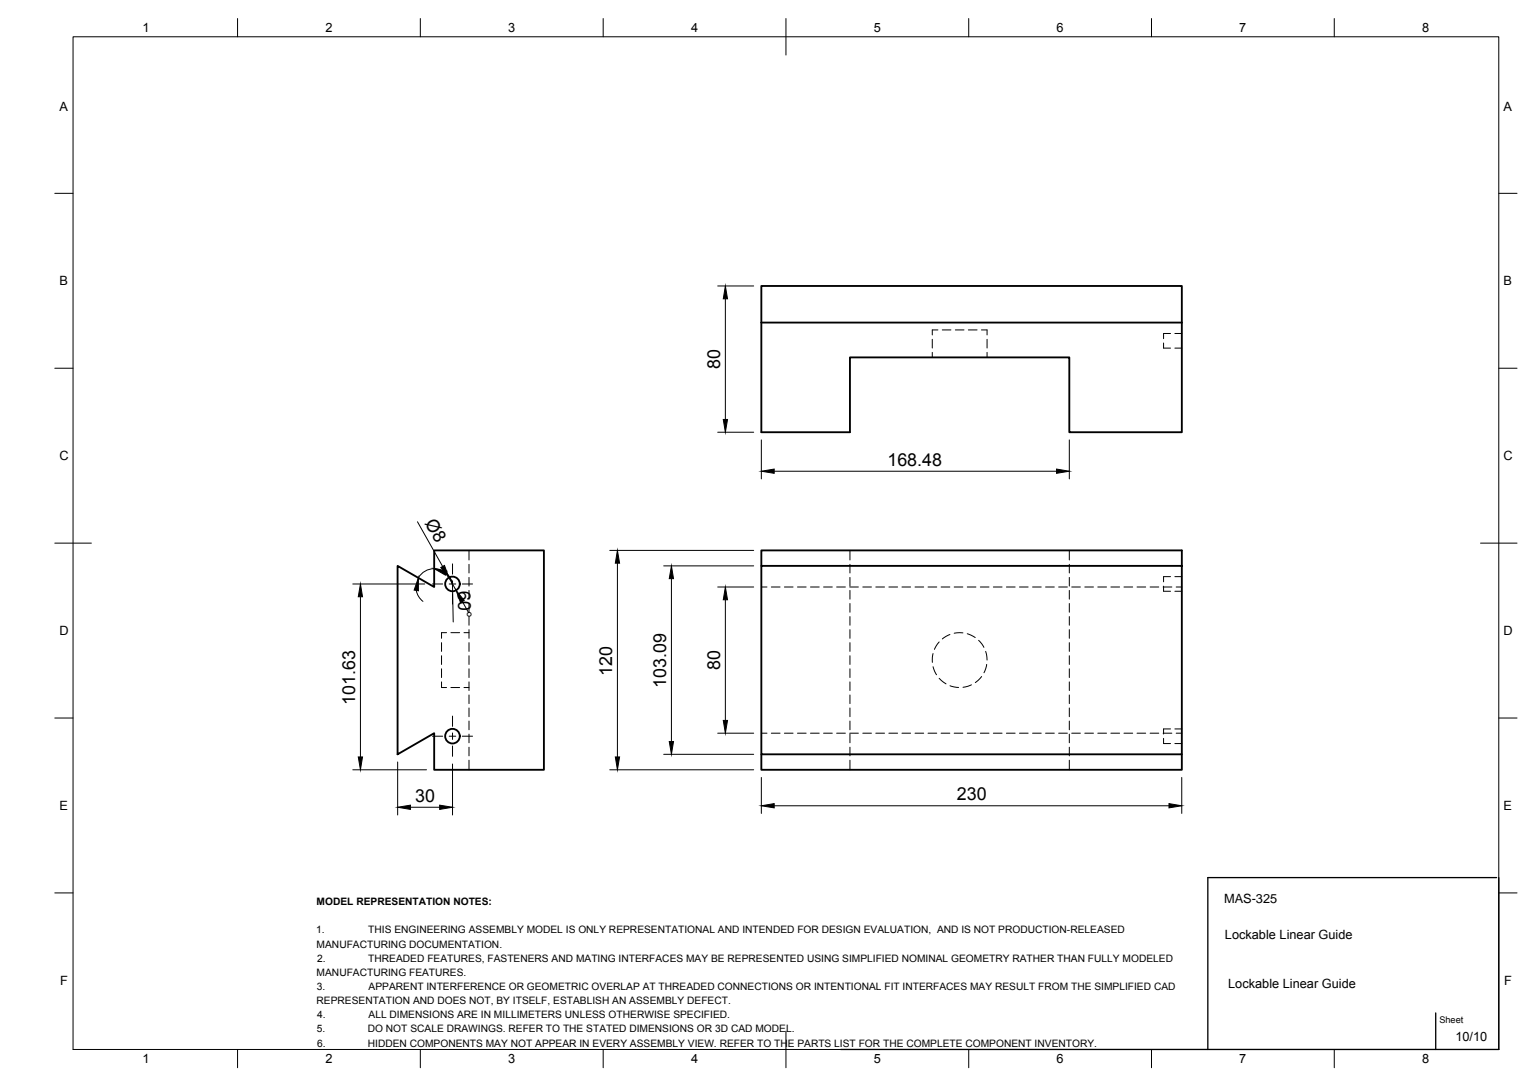
ISO-10303-21;
HEADER;
FILE_DESCRIPTION (('STEP AP214'),
    '1' );
FILE_NAME ('Lockable Linear Guide.step',
    '2026-10-08T01:23:29',
    ( '' ),
    ( '' ),
    'SwSTEP 2.0',
    'SolidWorks 2025',
    '' );
FILE_SCHEMA (( 'AUTOMOTIVE_DESIGN' ));
ENDSEC;

DATA;
#90=ORIENTED_EDGE ( 'NONE', *, *, #2858, .T. ) ;
#132=EDGE_LOOP ( 'NONE', ( #26426, #7526, #45933, #33902, #50296, #18073, #41197, #48921 ) ) ;
#156=DIRECTION ( 'NONE',  ( -1.000000000000000000, 0.000000000000000000, 0.000000000000000000 ) ) ;
#179=CIRCLE ( 'NONE', #49719, 4.000000000000003553 ) ;
#250=EDGE_CURVE ( 'NONE', #5889, #26611, #27078, .T. ) ;
#277=CARTESIAN_POINT ( 'NONE',  ( -108.4791267515088435, -173.5000000000000284, 60.00000000000002132 ) ) ;
#336=CARTESIAN_POINT ( 'NONE',  ( -170.0000000000000284, -123.5000000000000284, 41.63467731922665394 ) ) ;
#443=AXIS2_PLACEMENT_3D ( 'NONE', #25570, #1406, #41340 ) ;
#636=VECTOR ( 'NONE', #32808, 1000.000000000000000 ) ;
#695=DIRECTION ( 'NONE',  ( -1.000000000000000000, -0.000000000000000000, -0.000000000000000000 ) ) ;
#704=DIRECTION ( 'NONE',  ( 0.000000000000000000, 0.000000000000000000, 1.000000000000000000 ) ) ;
#786=FACE_OUTER_BOUND ( 'NONE', #39466, .T. ) ;
#796=ORIENTED_EDGE ( 'NONE', *, *, #49816, .F. ) ;
#802=PRODUCT ( 'Lockable Linear Guide', 'Lockable Linear Guide', '', ( #17073 ) ) ;
#812=ORIENTED_EDGE ( 'NONE', *, *, #27131, .F. ) ;
#837=CARTESIAN_POINT ( 'NONE',  ( -108.4791267515088435, -173.5000000000000284, -186.7953921478704729 ) ) ;
#930=ORIENTED_EDGE ( 'NONE', *, *, #25942, .T. ) ;
#1037=CARTESIAN_POINT ( 'NONE',  ( -48.47912675150885065, -132.5479369270331915, -14.99999999999999289 ) ) ;
#1384=DIRECTION ( 'NONE',  ( 0.000000000000000000, -0.000000000000000000, -1.000000000000000000 ) ) ;
#1394=ORIENTED_EDGE ( 'NONE', *, *, #30188, .F. ) ;
#1406=DIRECTION ( 'NONE',  ( -1.000000000000000000, -0.000000000000000000, -0.000000000000000000 ) ) ;
#1447=ORIENTED_EDGE ( 'NONE', *, *, #35273, .F. ) ;
#1451=VECTOR ( 'NONE', #28447, 1000.000000000000000 ) ;
#1479=PLANE ( 'NONE',  #26156 ) ;
#1584=ORIENTED_EDGE ( 'NONE', *, *, #16405, .F. ) ;
#1612=EDGE_LOOP ( 'NONE', ( #12933, #1584, #930, #8824 ) ) ;
#1633=LINE ( 'NONE', #10286, #39618 ) ;
#1706=ORIENTED_EDGE ( 'NONE', *, *, #8640, .T. ) ;
#1807=VERTEX_POINT ( 'NONE', #30021 ) ;
#1816=ADVANCED_FACE ( 'NONE', ( #26588 ), #46575, .T. ) ;
#1817=CARTESIAN_POINT ( 'NONE',  ( 11.52087324849114580, -173.5000000000000284, 60.00000000000002132 ) ) ;
#1925=FACE_OUTER_BOUND ( 'NONE', #13673, .T. ) ;
#1976=LINE ( 'NONE', #21175, #2305 ) ;
#1993=CARTESIAN_POINT ( 'NONE',  ( 60.00000000000001421, -173.5000000000000284, -60.00000000000001421 ) ) ;
#2056=DIRECTION ( 'NONE',  ( 0.000000000000000000, -1.000000000000000000, -1.156482317317871232E-16 ) ) ;
#2228=AXIS2_PLACEMENT_3D ( 'NONE', #10978, #49900, #2056 ) ;
#2305=VECTOR ( 'NONE', #5936, 1000.000000000000227 ) ;
#2339=ORIENTED_EDGE ( 'NONE', *, *, #30188, .T. ) ;
#2425=ORIENTED_EDGE ( 'NONE', *, *, #7091, .T. ) ;
#2440=AXIS2_PLACEMENT_3D ( 'NONE', #20656, #695, #36165 ) ;
#2504=VECTOR ( 'NONE', #19863, 1000.000000000000000 ) ;
#2563=LINE ( 'NONE', #30161, #47203 ) ;
#2579=VERTEX_POINT ( 'NONE', #42225 ) ;
#2728=AXIS2_PLACEMENT_3D ( 'NONE', #8668, #20762, #36793 ) ;
#2858=EDGE_CURVE ( 'NONE', #12202, #25229, #23144, .T. ) ;
#2997=CARTESIAN_POINT ( 'NONE',  ( -170.0000000000000284, -123.5000000000000284, -41.63467731922663972 ) ) ;
#3011=ADVANCED_FACE ( 'NONE', ( #21172 ), #41397, .T. ) ;
#3040=AXIS2_PLACEMENT_3D ( 'NONE', #8328, #24354, #704 ) ;
#3126=CARTESIAN_POINT ( 'NONE',  ( -48.47912675150885065, -117.5479369270332057, 6.938893903907228378E-15 ) ) ;
#3149=FACE_OUTER_BOUND ( 'NONE', #40264, .T. ) ;
#3357=ORIENTED_EDGE ( 'NONE', *, *, #51024, .F. ) ;
#3379=DIRECTION ( 'NONE',  ( 0.000000000000000000, 0.000000000000000000, -1.000000000000000000 ) ) ;
#3534=ADVANCED_FACE ( 'NONE', ( #40171 ), #8119, .F. ) ;
#3586=DIRECTION ( 'NONE',  ( 0.000000000000000000, 0.000000000000000000, 1.000000000000000000 ) ) ;
#3669=ORIENTED_EDGE ( 'NONE', *, *, #2858, .F. ) ;
#3702=EDGE_CURVE ( 'NONE', #25229, #12202, #41772, .T. ) ;
#3714=CARTESIAN_POINT ( 'NONE',  ( 0.000000000000000000, 0.000000000000000000, 0.000000000000000000 ) ) ;
#3839=LINE ( 'NONE', #32206, #2504 ) ;
#3884=ADVANCED_FACE ( 'NONE', ( #18845 ), #19624, .F. ) ;
#4042=DIRECTION ( 'NONE',  ( -1.000000000000000000, 0.000000000000000000, 0.000000000000000000 ) ) ;
#4117=DIRECTION ( 'NONE',  ( -0.000000000000000000, 1.000000000000000000, 0.000000000000000000 ) ) ;
#4436=AXIS2_PLACEMENT_3D ( 'NONE', #27266, #23079, #39090 ) ;
#4450=SHAPE_DEFINITION_REPRESENTATION ( #50801, #40181 ) ;
#4565=CARTESIAN_POINT ( 'NONE',  ( -170.0000000000000284, -113.5000000000000142, -60.00000000000001421 ) ) ;
#4624=LINE ( 'NONE', #16739, #41748 ) ;
#4697=DIRECTION ( 'NONE',  ( 1.000000000000000000, -0.000000000000000000, 0.000000000000000000 ) ) ;
#4803=ADVANCED_FACE ( 'NONE', ( #30178 ), #22026, .F. ) ;
#5081=EDGE_CURVE ( 'NONE', #39780, #15096, #51717, .T. ) ;
#5204=APPLICATION_CONTEXT ( 'automotive_design' ) ;
#5290=CARTESIAN_POINT ( 'NONE',  ( -160.0000000000000284, -123.5000000000000284, 37.63467731922665394 ) ) ;
#5334=EDGE_CURVE ( 'NONE', #50561, #45007, #21125, .T. ) ;
#5347=ORIENTED_EDGE ( 'NONE', *, *, #41312, .T. ) ;
#5499=DIRECTION ( 'NONE',  ( 0.000000000000000000, 0.000000000000000000, 1.000000000000000000 ) ) ;
#5755=DIRECTION ( 'NONE',  ( -0.000000000000000000, 1.000000000000000000, 0.000000000000000000 ) ) ;
#5889=VERTEX_POINT ( 'NONE', #13449 ) ;
#5920=CARTESIAN_POINT ( 'NONE',  ( -170.0000000000000284, -113.5000000000000000, 60.00000000000000711 ) ) ;
#5936=DIRECTION ( 'NONE',  ( 0.000000000000000000, 0.8660254037844354880, -0.5000000000000054401 ) ) ;
#5939=CARTESIAN_POINT ( 'NONE',  ( -170.0000000000000284, -93.50000000000002842, 51.54700538379266561 ) ) ;
#6074=DIRECTION ( 'NONE',  ( 0.000000000000000000, 1.000000000000000000, -6.938893903907222461E-16 ) ) ;
#6250=CARTESIAN_POINT ( 'NONE',  ( -48.47912675150885065, -132.5479369270331915, 15.00000000000000711 ) ) ;
#6266=LINE ( 'NONE', #29651, #12782 ) ;
#6291=VECTOR ( 'NONE', #44469, 1000.000000000000000 ) ;
#6492=AXIS2_PLACEMENT_3D ( 'NONE', #10560, #37378, #1384 ) ;
#6556=CARTESIAN_POINT ( 'NONE',  ( -170.0000000000000284, -93.50000000000001421, -51.54700538379269403 ) ) ;
#6621=PRODUCT_DEFINITION_FORMATION_WITH_SPECIFIED_SOURCE ( 'ANY', '', #802, .NOT_KNOWN. ) ;
#6666=CARTESIAN_POINT ( 'NONE',  ( 60.00000000000001421, -93.50000000000002842, 51.54700538379266561 ) ) ;
#6722=DIRECTION ( 'NONE',  ( 0.000000000000000000, 0.000000000000000000, -1.000000000000000000 ) ) ;
#6739=VERTEX_POINT ( 'NONE', #23218 ) ;
#6761=ORIENTED_EDGE ( 'NONE', *, *, #34984, .F. ) ;
#6778=ORIENTED_EDGE ( 'NONE', *, *, #35273, .T. ) ;
#6884=CIRCLE ( 'NONE', #13595, 4.000000000000003553 ) ;
#7009=LINE ( 'NONE', #10691, #40460 ) ;
#7091=EDGE_CURVE ( 'NONE', #43619, #46084, #1633, .T. ) ;
#7274=VECTOR ( 'NONE', #21684, 1000.000000000000000 ) ;
#7325=EDGE_CURVE ( 'NONE', #21917, #22206, #27850, .T. ) ;
#7393=ADVANCED_FACE ( 'NONE', ( #786 ), #44423, .F. ) ;
#7446=STYLED_ITEM ( 'NONE', ( #27799 ), #36582 ) ;
#7526=ORIENTED_EDGE ( 'NONE', *, *, #12854, .T. ) ;
#7530=LINE ( 'NONE', #39563, #51990 ) ;
#7608=CARTESIAN_POINT ( 'NONE',  ( -48.47912675150885065, -132.5479369270331915, 6.938893903907228378E-15 ) ) ;
#7629=PLANE ( 'NONE',  #15354 ) ;
#7670=EDGE_CURVE ( 'NONE', #21917, #37982, #47012, .T. ) ;
#7675=EDGE_CURVE ( 'NONE', #6739, #36835, #47273, .T. ) ;
#7689=CARTESIAN_POINT ( 'NONE',  ( -108.4791267515088435, -173.5000000000000284, -60.00000000000002842 ) ) ;
#7786=ORIENTED_EDGE ( 'NONE', *, *, #39934, .F. ) ;
#7864=( NAMED_UNIT ( * ) SI_UNIT ( $, .STERADIAN. ) SOLID_ANGLE_UNIT ( ) );
#8032=ORIENTED_EDGE ( 'NONE', *, *, #20852, .F. ) ;
#8119=PLANE ( 'NONE',  #19926 ) ;
#8136=PLANE ( 'NONE',  #21291 ) ;
#8210=LINE ( 'NONE', #32116, #16954 ) ;
#8211=LINE ( 'NONE', #24246, #23898 ) ;
#8256=( GEOMETRIC_REPRESENTATION_CONTEXT ( 3 ) GLOBAL_UNCERTAINTY_ASSIGNED_CONTEXT ( ( #38494 ) ) GLOBAL_UNIT_ASSIGNED_CONTEXT ( ( #51007, #48078, #7864 ) ) REPRESENTATION_CONTEXT ( 'NONE', 'WORKASPACE' ) );
#8328=CARTESIAN_POINT ( 'NONE',  ( -160.0000000000000284, -123.5000000000000284, 41.63467731922665394 ) ) ;
#8335=ORIENTED_EDGE ( 'NONE', *, *, #40361, .T. ) ;
#8419=VECTOR ( 'NONE', #46643, 1000.000000000000000 ) ;
#8438=DIRECTION ( 'NONE',  ( 1.000000000000000000, 0.000000000000000000, 0.000000000000000000 ) ) ;
#8607=CARTESIAN_POINT ( 'NONE',  ( -170.0000000000000284, -173.5000000000000284, 60.00000000000000000 ) ) ;
#8640=EDGE_CURVE ( 'NONE', #34090, #37367, #6266, .T. ) ;
#8668=CARTESIAN_POINT ( 'NONE',  ( -48.47912675150885065, -117.5479369270332057, 6.938893903907228378E-15 ) ) ;
#8726=CIRCLE ( 'NONE', #26365, 4.000000000000003553 ) ;
#8824=ORIENTED_EDGE ( 'NONE', *, *, #28783, .T. ) ;
#8898=AXIS2_PLACEMENT_3D ( 'NONE', #49637, #26216, #5499 ) ;
#9113=DIRECTION ( 'NONE',  ( 0.000000000000000000, 1.000000000000000000, -6.938893903907229364E-16 ) ) ;
#9210=ORIENTED_EDGE ( 'NONE', *, *, #26761, .T. ) ;
#9235=CARTESIAN_POINT ( 'NONE',  ( 60.00000000000001421, -113.5000000000000142, 39.99999999999998579 ) ) ;
#9343=DIRECTION ( 'NONE',  ( 0.000000000000000000, 0.000000000000000000, 1.000000000000000000 ) ) ;
#9599=FACE_OUTER_BOUND ( 'NONE', #18883, .T. ) ;
#9606=DIRECTION ( 'NONE',  ( 0.000000000000000000, -0.000000000000000000, -1.000000000000000000 ) ) ;
#9641=CARTESIAN_POINT ( 'NONE',  ( 11.52087324849114580, -132.5479369270331915, 60.00000000000002132 ) ) ;
#9692=DIRECTION ( 'NONE',  ( 0.000000000000000000, 0.000000000000000000, 1.000000000000000000 ) ) ;
#9707=LINE ( 'NONE', #46242, #16121 ) ;
#9873=PLANE ( 'NONE',  #51406 ) ;
#9886=CARTESIAN_POINT ( 'NONE',  ( -170.0000000000000284, -173.5000000000000284, -60.00000000000001421 ) ) ;
#9890=CARTESIAN_POINT ( 'NONE',  ( -48.47912675150885065, -117.5479369270332057, -14.99999999999999289 ) ) ;
#9894=FACE_OUTER_BOUND ( 'NONE', #13604, .T. ) ;
#9950=DIRECTION ( 'NONE',  ( -1.000000000000000000, -0.000000000000000000, -0.000000000000000000 ) ) ;
#9970=( GEOMETRIC_REPRESENTATION_CONTEXT ( 3 ) GLOBAL_UNCERTAINTY_ASSIGNED_CONTEXT ( ( #42696 ) ) GLOBAL_UNIT_ASSIGNED_CONTEXT ( ( #32535, #11255, #51743 ) ) REPRESENTATION_CONTEXT ( 'NONE', 'WORKASPACE' ) );
#10106=CARTESIAN_POINT ( 'NONE',  ( -170.0000000000000284, -173.5000000000000284, -60.00000000000001421 ) ) ;
#10203=CARTESIAN_POINT ( 'NONE',  ( 11.52087324849114580, -132.5479369270331915, -60.00000000000002842 ) ) ;
#10286=CARTESIAN_POINT ( 'NONE',  ( -108.4791267515088435, -132.5479369270331915, -186.7953921478704729 ) ) ;
#10356=EDGE_LOOP ( 'NONE', ( #24313, #24164, #49378, #34675, #49345, #52015, #40532, #11783 ) ) ;
#10451=EDGE_CURVE ( 'NONE', #40019, #43044, #20726, .T. ) ;
#10560=CARTESIAN_POINT ( 'NONE',  ( -170.0000000000000284, -173.5000000000000284, 60.00000000000000000 ) ) ;
#10624=ORIENTED_EDGE ( 'NONE', *, *, #12854, .F. ) ;
#10691=CARTESIAN_POINT ( 'NONE',  ( 11.52087324849114580, -173.5000000000000284, -60.00000000000002842 ) ) ;
#10978=CARTESIAN_POINT ( 'NONE',  ( -170.0000000000000284, -113.5000000000000000, 60.00000000000000711 ) ) ;
#11043=DIRECTION ( 'NONE',  ( -0.000000000000000000, 0.000000000000000000, -1.000000000000000000 ) ) ;
#11073=LINE ( 'NONE', #43660, #36677 ) ;
#11182=EDGE_CURVE ( 'NONE', #15096, #5889, #41263, .T. ) ;
#11244=CARTESIAN_POINT ( 'NONE',  ( -160.0000000000000284, -123.5000000000000284, -45.63467731922664683 ) ) ;
#11255=( NAMED_UNIT ( * ) PLANE_ANGLE_UNIT ( ) SI_UNIT ( $, .RADIAN. ) );
#11377=AXIS2_PLACEMENT_3D ( 'NONE', #45125, #9113, #25142 ) ;
#11550=DIRECTION ( 'NONE',  ( 0.000000000000000000, 0.000000000000000000, 1.000000000000000000 ) ) ;
#11559=CARTESIAN_POINT ( 'NONE',  ( -170.0000000000000284, -113.5000000000000000, -40.00000000000001421 ) ) ;
#11783=ORIENTED_EDGE ( 'NONE', *, *, #18126, .F. ) ;
#11973=ADVANCED_FACE ( 'NONE', ( #31963 ), #24595, .F. ) ;
#11980=FACE_OUTER_BOUND ( 'NONE', #14534, .T. ) ;
#12079=ORIENTED_EDGE ( 'NONE', *, *, #7670, .F. ) ;
#12151=ADVANCED_FACE ( 'NONE', ( #33780 ), #14082, .T. ) ;
#12171=ORIENTED_EDGE ( 'NONE', *, *, #27174, .T. ) ;
#12202=VERTEX_POINT ( 'NONE', #47174 ) ;
#12279=ORIENTED_EDGE ( 'NONE', *, *, #8640, .F. ) ;
#12368=LINE ( 'NONE', #24456, #15745 ) ;
#12399=VECTOR ( 'NONE', #21306, 1000.000000000000000 ) ;
#12503=VECTOR ( 'NONE', #29419, 1000.000000000000000 ) ;
#12529=ORIENTED_EDGE ( 'NONE', *, *, #26739, .F. ) ;
#12534=ORIENTED_EDGE ( 'NONE', *, *, #48332, .F. ) ;
#12539=CARTESIAN_POINT ( 'NONE',  ( -108.4791267515088435, -132.5479369270331915, -60.00000000000002842 ) ) ;
#12593=ORIENTED_EDGE ( 'NONE', *, *, #31408, .F. ) ;
#12782=VECTOR ( 'NONE', #42516, 1000.000000000000000 ) ;
#12783=AXIS2_PLACEMENT_3D ( 'NONE', #2997, #19039, #35065 ) ;
#12854=EDGE_CURVE ( 'NONE', #19578, #22206, #40332, .T. ) ;
#12933=ORIENTED_EDGE ( 'NONE', *, *, #43822, .F. ) ;
#12967=EDGE_CURVE ( 'NONE', #12202, #41381, #3839, .T. ) ;
#12969=ADVANCED_BREP_SHAPE_REPRESENTATION ( '', ( #36582, #31742 ), #8256 ) ;
#12978=CARTESIAN_POINT ( 'NONE',  ( 11.52087324849114580, -173.5000000000000284, -60.00000000000002842 ) ) ;
#13096=ORIENTED_EDGE ( 'NONE', *, *, #22634, .T. ) ;
#13139=EDGE_CURVE ( 'NONE', #37982, #2579, #14846, .T. ) ;
#13449=CARTESIAN_POINT ( 'NONE',  ( -170.0000000000000284, -123.5000000000000284, 37.63467731922665394 ) ) ;
#13595=AXIS2_PLACEMENT_3D ( 'NONE', #37606, #49177, #21314 ) ;
#13600=CARTESIAN_POINT ( 'NONE',  ( -170.0000000000000284, -123.5000000000000284, -45.63467731922664683 ) ) ;
#13604=EDGE_LOOP ( 'NONE', ( #5347, #38768, #49800, #12529 ) ) ;
#13673=EDGE_LOOP ( 'NONE', ( #38678, #41141, #40067, #8335 ) ) ;
#13697=VECTOR ( 'NONE', #27014, 1000.000000000000000 ) ;
#13767=CARTESIAN_POINT ( 'NONE',  ( 60.00000000000001421, 0.000000000000000000, 0.000000000000000000 ) ) ;
#13816=DIRECTION ( 'NONE',  ( -0.000000000000000000, 1.000000000000000000, 1.346129392433909288E-16 ) ) ;
#13831=DIRECTION ( 'NONE',  ( 0.000000000000000000, -0.000000000000000000, 1.000000000000000000 ) ) ;
#13911=DIRECTION ( 'NONE',  ( 0.000000000000000000, -1.000000000000000000, -1.156482317317871232E-16 ) ) ;
#14082=PLANE ( 'NONE',  #30148 ) ;
#14120=ADVANCED_FACE ( 'NONE', ( #46766 ), #23368, .F. ) ;
#14343=VECTOR ( 'NONE', #49551, 1000.000000000000000 ) ;
#14444=ORIENTED_EDGE ( 'NONE', *, *, #7325, .T. ) ;
#14534=EDGE_LOOP ( 'NONE', ( #15913, #47480 ) ) ;
#14550=DIRECTION ( 'NONE',  ( 0.000000000000000000, -0.8660254037844354880, -0.5000000000000054401 ) ) ;
#14846=LINE ( 'NONE', #45863, #8419 ) ;
#14996=COLOUR_RGB ( '', 0.31764706, 0.68627451, 0.89019608) ;
#15096=VERTEX_POINT ( 'NONE', #21880 ) ;
#15234=ORIENTED_EDGE ( 'NONE', *, *, #15999, .F. ) ;
#15253=CARTESIAN_POINT ( 'NONE',  ( 60.00000000000001421, -113.5000000000000142, -60.00000000000001421 ) ) ;
#15260=VECTOR ( 'NONE', #41553, 1000.000000000000000 ) ;
#15315=VERTEX_POINT ( 'NONE', #8607 ) ;
#15354=AXIS2_PLACEMENT_3D ( 'NONE', #47066, #23650, #11043 ) ;
#15408=EDGE_CURVE ( 'NONE', #6739, #40019, #8726, .T. ) ;
#15481=SURFACE_STYLE_USAGE ( .BOTH. , #35429 ) ;
#15677=DIRECTION ( 'NONE',  ( 0.000000000000000000, 0.8660254037844354880, -0.5000000000000054401 ) ) ;
#15732=EDGE_LOOP ( 'NONE', ( #35257, #38291, #24666, #18404 ) ) ;
#15745=VECTOR ( 'NONE', #41261, 1000.000000000000000 ) ;
#15797=ORIENTED_EDGE ( 'NONE', *, *, #20852, .T. ) ;
#15870=ORIENTED_EDGE ( 'NONE', *, *, #25942, .F. ) ;
#15913=ORIENTED_EDGE ( 'NONE', *, *, #5081, .T. ) ;
#15999=EDGE_CURVE ( 'NONE', #43044, #36835, #46598, .T. ) ;
#16000=FILL_AREA_STYLE ('',( #32007 ) ) ;
#16121=VECTOR ( 'NONE', #13911, 1000.000000000000000 ) ;
#16154=CARTESIAN_POINT ( 'NONE',  ( -170.0000000000000284, -123.5000000000000284, -37.63467731922663972 ) ) ;
#16267=ORIENTED_EDGE ( 'NONE', *, *, #25688, .F. ) ;
#16347=EDGE_CURVE ( 'NONE', #39780, #26611, #21887, .T. ) ;
#16405=EDGE_CURVE ( 'NONE', #51701, #45007, #35498, .T. ) ;
#16523=VERTEX_POINT ( 'NONE', #277 ) ;
#16627=LINE ( 'NONE', #22038, #6291 ) ;
#16693=DIRECTION ( 'NONE',  ( 0.000000000000000000, 1.000000000000000000, 0.000000000000000000 ) ) ;
#16723=CARTESIAN_POINT ( 'NONE',  ( 60.00000000000001421, -93.50000000000001421, -51.54700538379269403 ) ) ;
#16739=CARTESIAN_POINT ( 'NONE',  ( 11.52087324849114580, -173.5000000000000284, -186.7953921478704729 ) ) ;
#16778=VECTOR ( 'NONE', #15677, 1000.000000000000227 ) ;
#16931=ORIENTED_EDGE ( 'NONE', *, *, #48077, .T. ) ;
#16954=VECTOR ( 'NONE', #48161, 1000.000000000000000 ) ;
#16998=PLANE ( 'NONE',  #11377 ) ;
#17073=PRODUCT_CONTEXT ( 'NONE', #44796, 'mechanical' ) ;
#17149=CARTESIAN_POINT ( 'NONE',  ( -170.0000000000000284, -113.5000000000000000, -40.00000000000001421 ) ) ;
#17222=CARTESIAN_POINT ( 'NONE',  ( 60.00000000000001421, -113.5000000000000000, 60.00000000000000711 ) ) ;
#17509=CARTESIAN_POINT ( 'NONE',  ( -170.0000000000000284, -173.5000000000000284, 60.00000000000000000 ) ) ;
#17555=EDGE_LOOP ( 'NONE', ( #16931, #33943 ) ) ;
#17672=DIRECTION ( 'NONE',  ( -0.000000000000000000, -0.000000000000000000, 1.000000000000000000 ) ) ;
#17802=CARTESIAN_POINT ( 'NONE',  ( -160.0000000000000284, -123.5000000000000284, 45.63467731922665394 ) ) ;
#17839=DIRECTION ( 'NONE',  ( -0.000000000000000000, 1.000000000000000000, 0.000000000000000000 ) ) ;
#17887=ORIENTED_EDGE ( 'NONE', *, *, #13139, .T. ) ;
#17941=CARTESIAN_POINT ( 'NONE',  ( -160.0000000000000284, -123.5000000000000284, 45.63467731922665394 ) ) ;
#17998=LINE ( 'NONE', #5920, #14343 ) ;
#18016=ORIENTED_EDGE ( 'NONE', *, *, #32778, .F. ) ;
#18024=VERTEX_POINT ( 'NONE', #17222 ) ;
#18073=ORIENTED_EDGE ( 'NONE', *, *, #27742, .T. ) ;
#18126=EDGE_CURVE ( 'NONE', #31030, #50561, #37956, .T. ) ;
#18404=ORIENTED_EDGE ( 'NONE', *, *, #16347, .F. ) ;
#18716=ORIENTED_EDGE ( 'NONE', *, *, #18126, .T. ) ;
#18781=ORIENTED_EDGE ( 'NONE', *, *, #21374, .F. ) ;
#18842=DIRECTION ( 'NONE',  ( 0.000000000000000000, -1.000000000000000000, -1.156482317317871232E-16 ) ) ;
#18845=FACE_OUTER_BOUND ( 'NONE', #24892, .T. ) ;
#18883=EDGE_LOOP ( 'NONE', ( #43401, #39571, #49288, #42576 ) ) ;
#18922=AXIS2_PLACEMENT_3D ( 'NONE', #25563, #38162, #45812 ) ;
#18981=EDGE_LOOP ( 'NONE', ( #10624, #21725, #47715, #14444 ) ) ;
#19039=DIRECTION ( 'NONE',  ( -1.000000000000000000, 0.000000000000000000, 0.000000000000000000 ) ) ;
#19104=DIRECTION ( 'NONE',  ( 0.000000000000000000, 1.000000000000000000, 0.000000000000000000 ) ) ;
#19140=CARTESIAN_POINT ( 'NONE',  ( -170.0000000000000284, -123.5000000000000284, 45.63467731922665394 ) ) ;
#19141=EDGE_LOOP ( 'NONE', ( #51518, #41362 ) ) ;
#19429=CYLINDRICAL_SURFACE ( 'NONE', #42471, 4.000000000000003553 ) ;
#19472=DIRECTION ( 'NONE',  ( 1.000000000000000000, 0.000000000000000000, 0.000000000000000000 ) ) ;
#19578=VERTEX_POINT ( 'NONE', #50803 ) ;
#19624=PLANE ( 'NONE',  #35909 ) ;
#19675=ORIENTED_EDGE ( 'NONE', *, *, #51384, .F. ) ;
#19690=DIRECTION ( 'NONE',  ( 0.000000000000000000, -0.5000000000000054401, -0.8660254037844354880 ) ) ;
#19863=DIRECTION ( 'NONE',  ( 0.000000000000000000, -1.000000000000000000, 0.000000000000000000 ) ) ;
#19926=AXIS2_PLACEMENT_3D ( 'NONE', #48064, #4697, #24933 ) ;
#19981=DIRECTION ( 'NONE',  ( 1.000000000000000000, 0.000000000000000000, 0.000000000000000000 ) ) ;
#20119=CARTESIAN_POINT ( 'NONE',  ( 60.00000000000001421, -113.5000000000000000, -40.00000000000001421 ) ) ;
#20209=CARTESIAN_POINT ( 'NONE',  ( -170.0000000000000284, -113.5000000000000000, -40.00000000000001421 ) ) ;
#20214=DIRECTION ( 'NONE',  ( 0.000000000000000000, 0.000000000000000000, 1.000000000000000000 ) ) ;
#20385=CARTESIAN_POINT ( 'NONE',  ( -48.47912675150885065, -117.5479369270332057, 6.938893903907228378E-15 ) ) ;
#20656=CARTESIAN_POINT ( 'NONE',  ( -160.0000000000000284, -123.5000000000000284, 41.63467731922665394 ) ) ;
#20726=LINE ( 'NONE', #36759, #636 ) ;
#20762=DIRECTION ( 'NONE',  ( 0.000000000000000000, -1.000000000000000000, 0.000000000000000000 ) ) ;
#20852=EDGE_CURVE ( 'NONE', #37982, #24439, #11073, .T. ) ;
#20887=DIRECTION ( 'NONE',  ( -0.000000000000000000, 0.000000000000000000, -1.000000000000000000 ) ) ;
#20941=FACE_OUTER_BOUND ( 'NONE', #1612, .T. ) ;
#21009=CARTESIAN_POINT ( 'NONE',  ( -170.0000000000000284, -173.5000000000000284, 60.00000000000000000 ) ) ;
#21023=CARTESIAN_POINT ( 'NONE',  ( -170.0000000000000284, -93.50000000000002842, 51.54700538379266561 ) ) ;
#21030=CARTESIAN_POINT ( 'NONE',  ( -170.0000000000000284, -173.5000000000000284, 60.00000000000000000 ) ) ;
#21079=DIRECTION ( 'NONE',  ( 1.000000000000000000, 0.000000000000000000, 0.000000000000000000 ) ) ;
#21125=LINE ( 'NONE', #31915, #42509 ) ;
#21169=ADVANCED_FACE ( 'NONE', ( #11980 ), #32218, .T. ) ;
#21172=FACE_OUTER_BOUND ( 'NONE', #21730, .T. ) ;
#21175=CARTESIAN_POINT ( 'NONE',  ( -170.0000000000000284, -113.5000000000000000, -40.00000000000001421 ) ) ;
#21210=CLOSED_SHELL ( 'NONE', ( #7393, #11973, #48689, #3011, #25257, #42751, #1816, #50114, #33355, #41780, #12151, #46137, #40465, #29791, #3534, #50466, #4803, #40061, #41032, #49219, #21169, #14120, #3884 ) ) ;
#21291=AXIS2_PLACEMENT_3D ( 'NONE', #11559, #19690, #36238 ) ;
#21296=ORIENTED_EDGE ( 'NONE', *, *, #26761, .F. ) ;
#21306=DIRECTION ( 'NONE',  ( -1.000000000000000000, -0.000000000000000000, -0.000000000000000000 ) ) ;
#21314=DIRECTION ( 'NONE',  ( 0.000000000000000000, 0.000000000000000000, 1.000000000000000000 ) ) ;
#21335=CARTESIAN_POINT ( 'NONE',  ( -160.0000000000000284, -123.5000000000000284, -41.63467731922663972 ) ) ;
#21374=EDGE_CURVE ( 'NONE', #31030, #34090, #4624, .T. ) ;
#21423=VERTEX_POINT ( 'NONE', #44834 ) ;
#21431=CIRCLE ( 'NONE', #18922, 4.000000000000003553 ) ;
#21662=PLANE ( 'NONE',  #44853 ) ;
#21684=DIRECTION ( 'NONE',  ( 1.000000000000000000, 0.000000000000000000, 0.000000000000000000 ) ) ;
#21716=DIRECTION ( 'NONE',  ( -1.000000000000000000, 0.000000000000000000, -0.000000000000000000 ) ) ;
#21725=ORIENTED_EDGE ( 'NONE', *, *, #28783, .F. ) ;
#21730=EDGE_LOOP ( 'NONE', ( #18781, #18716, #6761, #21296 ) ) ;
#21770=DIRECTION ( 'NONE',  ( 0.000000000000000000, 0.000000000000000000, 1.000000000000000000 ) ) ;
#21880=CARTESIAN_POINT ( 'NONE',  ( -160.0000000000000284, -123.5000000000000284, 37.63467731922665394 ) ) ;
#21887=LINE ( 'NONE', #17941, #36477 ) ;
#21917=VERTEX_POINT ( 'NONE', #42115 ) ;
#21944=ORIENTED_EDGE ( 'NONE', *, *, #40290, .T. ) ;
#21953=DIRECTION ( 'NONE',  ( 0.000000000000000000, -0.5000000000000054401, 0.8660254037844354880 ) ) ;
#22026=PLANE ( 'NONE',  #8898 ) ;
#22038=CARTESIAN_POINT ( 'NONE',  ( -48.47912675150885065, -117.5479369270332057, -14.99999999999999289 ) ) ;
#22206=VERTEX_POINT ( 'NONE', #16723 ) ;
#22303=AXIS2_PLACEMENT_3D ( 'NONE', #17509, #33525, #9606 ) ;
#22330=VECTOR ( 'NONE', #32826, 1000.000000000000000 ) ;
#22565=EDGE_LOOP ( 'NONE', ( #12279, #9210, #33239, #49745, #23246, #29973, #796, #50408 ) ) ;
#22634=EDGE_CURVE ( 'NONE', #24439, #26043, #31883, .T. ) ;
#22648=DIRECTION ( 'NONE',  ( 0.000000000000000000, 0.000000000000000000, -1.000000000000000000 ) ) ;
#23079=DIRECTION ( 'NONE',  ( -1.000000000000000000, 0.000000000000000000, 0.000000000000000000 ) ) ;
#23136=SHAPE_REPRESENTATION_RELATIONSHIP ( 'NONE' , 'NONE' ,  #40181, #12969 ) ;
#23144=CIRCLE ( 'NONE', #43230, 15.00000000000000000 ) ;
#23149=ORIENTED_EDGE ( 'NONE', *, *, #15408, .F. ) ;
#23218=CARTESIAN_POINT ( 'NONE',  ( -160.0000000000000284, -123.5000000000000284, -45.63467731922664683 ) ) ;
#23246=ORIENTED_EDGE ( 'NONE', *, *, #41378, .T. ) ;
#23368=CYLINDRICAL_SURFACE ( 'NONE', #43239, 15.00000000000000000 ) ;
#23650=DIRECTION ( 'NONE',  ( 1.000000000000000000, 0.000000000000000000, -0.000000000000000000 ) ) ;
#23710=CARTESIAN_POINT ( 'NONE',  ( -170.0000000000000284, -113.5000000000000142, -60.00000000000001421 ) ) ;
#23898=VECTOR ( 'NONE', #47384, 1000.000000000000000 ) ;
#23909=CARTESIAN_POINT ( 'NONE',  ( -170.0000000000000284, -93.50000000000001421, -51.54700538379269403 ) ) ;
#24094=EDGE_LOOP ( 'NONE', ( #2425, #25932, #27736, #38020 ) ) ;
#24164=ORIENTED_EDGE ( 'NONE', *, *, #26739, .T. ) ;
#24175=CARTESIAN_POINT ( 'NONE',  ( -108.4791267515088435, -173.5000000000000284, 60.00000000000002132 ) ) ;
#24246=CARTESIAN_POINT ( 'NONE',  ( -108.4791267515088435, -173.5000000000000284, -60.00000000000002842 ) ) ;
#24313=ORIENTED_EDGE ( 'NONE', *, *, #39934, .T. ) ;
#24335=DIRECTION ( 'NONE',  ( 0.000000000000000000, 0.000000000000000000, 1.000000000000000000 ) ) ;
#24354=DIRECTION ( 'NONE',  ( -1.000000000000000000, 0.000000000000000000, 0.000000000000000000 ) ) ;
#24439=VERTEX_POINT ( 'NONE', #44546 ) ;
#24456=CARTESIAN_POINT ( 'NONE',  ( -170.0000000000000284, -173.5000000000000284, -60.00000000000001421 ) ) ;
#24487=DIRECTION ( 'NONE',  ( 0.000000000000000000, 0.000000000000000000, 1.000000000000000000 ) ) ;
#24506=ORIENTED_EDGE ( 'NONE', *, *, #38897, .T. ) ;
#24595=CYLINDRICAL_SURFACE ( 'NONE', #2440, 4.000000000000003553 ) ;
#24666=ORIENTED_EDGE ( 'NONE', *, *, #250, .T. ) ;
#24888=LINE ( 'NONE', #44352, #37876 ) ;
#24892=EDGE_LOOP ( 'NONE', ( #41843, #3669 ) ) ;
#24933=DIRECTION ( 'NONE',  ( 0.000000000000000000, 0.000000000000000000, -1.000000000000000000 ) ) ;
#25142=DIRECTION ( 'NONE',  ( 0.000000000000000000, 6.938893903907229364E-16, 1.000000000000000000 ) ) ;
#25229=VERTEX_POINT ( 'NONE', #9890 ) ;
#25257=ADVANCED_FACE ( 'NONE', ( #20941 ), #16998, .T. ) ;
#25423=EDGE_LOOP ( 'NONE', ( #12171, #18016, #6778, #27155 ) ) ;
#25524=CARTESIAN_POINT ( 'NONE',  ( -170.0000000000000284, -113.5000000000000000, 60.00000000000000711 ) ) ;
#25563=CARTESIAN_POINT ( 'NONE',  ( -160.0000000000000284, -123.5000000000000284, -41.63467731922663972 ) ) ;
#25570=CARTESIAN_POINT ( 'NONE',  ( -160.0000000000000284, -123.5000000000000284, 41.63467731922665394 ) ) ;
#25579=FACE_OUTER_BOUND ( 'NONE', #132, .T. ) ;
#25688=EDGE_CURVE ( 'NONE', #2579, #31941, #50551, .T. ) ;
#25714=AXIS2_PLACEMENT_3D ( 'NONE', #27317, #6074, #46973 ) ;
#25776=DIRECTION ( 'NONE',  ( 0.000000000000000000, 6.938893903907222461E-16, 1.000000000000000000 ) ) ;
#25833=ORIENTED_EDGE ( 'NONE', *, *, #45658, .F. ) ;
#25914=PLANE ( 'NONE',  #49236 ) ;
#25932=ORIENTED_EDGE ( 'NONE', *, *, #49816, .T. ) ;
#25942=EDGE_CURVE ( 'NONE', #51701, #48674, #35525, .T. ) ;
#26043=VERTEX_POINT ( 'NONE', #25524 ) ;
#26156=AXIS2_PLACEMENT_3D ( 'NONE', #9886, #6722, #21716 ) ;
#26157=DIRECTION ( 'NONE',  ( -0.000000000000000000, 1.000000000000000000, 0.000000000000000000 ) ) ;
#26213=AXIS2_PLACEMENT_3D ( 'NONE', #34289, #45355, #9343 ) ;
#26216=DIRECTION ( 'NONE',  ( -1.000000000000000000, 0.000000000000000000, 0.000000000000000000 ) ) ;
#26365=AXIS2_PLACEMENT_3D ( 'NONE', #41965, #45413, #33045 ) ;
#26387=EDGE_LOOP ( 'NONE', ( #15234, #29531 ) ) ;
#26403=DIRECTION ( 'NONE',  ( 0.000000000000000000, -0.8660254037844354880, -0.5000000000000054401 ) ) ;
#26426=ORIENTED_EDGE ( 'NONE', *, *, #43822, .T. ) ;
#26588=FACE_OUTER_BOUND ( 'NONE', #25423, .T. ) ;
#26611=VERTEX_POINT ( 'NONE', #19140 ) ;
#26739=EDGE_CURVE ( 'NONE', #50099, #43619, #48815, .T. ) ;
#26761=EDGE_CURVE ( 'NONE', #34090, #1807, #24888, .T. ) ;
#26849=DIRECTION ( 'NONE',  ( 0.000000000000000000, -0.8660254037844354880, -0.5000000000000054401 ) ) ;
#27014=DIRECTION ( 'NONE',  ( 0.000000000000000000, -1.346129392433909288E-16, 1.000000000000000000 ) ) ;
#27078=CIRCLE ( 'NONE', #4436, 4.000000000000003553 ) ;
#27131=EDGE_CURVE ( 'NONE', #22206, #2579, #8210, .T. ) ;
#27155=ORIENTED_EDGE ( 'NONE', *, *, #35903, .T. ) ;
#27174=EDGE_CURVE ( 'NONE', #40951, #16523, #33436, .T. ) ;
#27266=CARTESIAN_POINT ( 'NONE',  ( -170.0000000000000284, -123.5000000000000284, 41.63467731922665394 ) ) ;
#27272=DIRECTION ( 'NONE',  ( -1.000000000000000000, -0.000000000000000000, -0.000000000000000000 ) ) ;
#27317=CARTESIAN_POINT ( 'NONE',  ( -170.0000000000000284, -113.5000000000000142, 39.99999999999998579 ) ) ;
#27601=FACE_BOUND ( 'NONE', #19141, .T. ) ;
#27736=ORIENTED_EDGE ( 'NONE', *, *, #27174, .F. ) ;
#27738=VECTOR ( 'NONE', #51851, 1000.000000000000000 ) ;
#27742=EDGE_CURVE ( 'NONE', #18024, #1807, #9707, .T. ) ;
#27799=PRESENTATION_STYLE_ASSIGNMENT (( #15481 ) ) ;
#27830=CARTESIAN_POINT ( 'NONE',  ( -108.4791267515088435, -132.5479369270331915, 60.00000000000000711 ) ) ;
#27850=LINE ( 'NONE', #23909, #48045 ) ;
#28278=DIRECTION ( 'NONE',  ( -0.000000000000000000, -0.000000000000000000, 1.000000000000000000 ) ) ;
#28447=DIRECTION ( 'NONE',  ( 0.000000000000000000, 6.938893903907222461E-16, 1.000000000000000000 ) ) ;
#28594=ORIENTED_EDGE ( 'NONE', *, *, #46249, .T. ) ;
#28783=EDGE_CURVE ( 'NONE', #48674, #19578, #37104, .T. ) ;
#28791=AXIS2_PLACEMENT_3D ( 'NONE', #21335, #33434, #24487 ) ;
#29419=DIRECTION ( 'NONE',  ( 0.000000000000000000, 0.000000000000000000, -1.000000000000000000 ) ) ;
#29531=ORIENTED_EDGE ( 'NONE', *, *, #40290, .F. ) ;
#29563=PRODUCT_DEFINITION_CONTEXT ( 'detailed design', #5204, 'design' ) ;
#29651=CARTESIAN_POINT ( 'NONE',  ( 11.52087324849114580, -173.5000000000000284, 60.00000000000002132 ) ) ;
#29694=ORIENTED_EDGE ( 'NONE', *, *, #22634, .F. ) ;
#29791=ADVANCED_FACE ( 'NONE', ( #25579 ), #21662, .T. ) ;
#29896=LINE ( 'NONE', #38034, #41411 ) ;
#29973=ORIENTED_EDGE ( 'NONE', *, *, #32778, .T. ) ;
#30004=AXIS2_PLACEMENT_3D ( 'NONE', #35641, #156, #3586 ) ;
#30021=CARTESIAN_POINT ( 'NONE',  ( 60.00000000000001421, -173.5000000000000284, 60.00000000000000000 ) ) ;
#30148=AXIS2_PLACEMENT_3D ( 'NONE', #45628, #13816, #34043 ) ;
#30161=CARTESIAN_POINT ( 'NONE',  ( 11.52087324849114580, -132.5479369270331915, -186.7953921478704729 ) ) ;
#30178=FACE_OUTER_BOUND ( 'NONE', #24094, .T. ) ;
#30188=EDGE_CURVE ( 'NONE', #25229, #38006, #16627, .T. ) ;
#30607=CIRCLE ( 'NONE', #44884, 15.00000000000000000 ) ;
#31020=FACE_OUTER_BOUND ( 'NONE', #48619, .T. ) ;
#31030=VERTEX_POINT ( 'NONE', #12978 ) ;
#31268=DIRECTION ( 'NONE',  ( 0.000000000000000000, 6.938893903907229364E-16, 1.000000000000000000 ) ) ;
#31273=VECTOR ( 'NONE', #27272, 1000.000000000000000 ) ;
#31385=CARTESIAN_POINT ( 'NONE',  ( -170.0000000000000284, -113.5000000000000142, 39.99999999999998579 ) ) ;
#31386=EDGE_CURVE ( 'NONE', #43619, #40951, #8211, .T. ) ;
#31408=EDGE_CURVE ( 'NONE', #41381, #38006, #30607, .T. ) ;
#31510=DIRECTION ( 'NONE',  ( -1.000000000000000000, -0.000000000000000000, -0.000000000000000000 ) ) ;
#31521=FACE_OUTER_BOUND ( 'NONE', #18981, .T. ) ;
#31524=ORIENTED_EDGE ( 'NONE', *, *, #3702, .T. ) ;
#31742=AXIS2_PLACEMENT_3D ( 'NONE', #3714, #31843, #8438 ) ;
#31843=DIRECTION ( 'NONE',  ( 0.000000000000000000, 0.000000000000000000, 1.000000000000000000 ) ) ;
#31883=LINE ( 'NONE', #39503, #1451 ) ;
#31915=CARTESIAN_POINT ( 'NONE',  ( 60.00000000000001421, -173.5000000000000284, -60.00000000000001421 ) ) ;
#31941=VERTEX_POINT ( 'NONE', #48010 ) ;
#31963=FACE_OUTER_BOUND ( 'NONE', #15732, .T. ) ;
#32007=FILL_AREA_STYLE_COLOUR ( '', #14996 ) ;
#32116=CARTESIAN_POINT ( 'NONE',  ( 60.00000000000001421, -93.50000000000001421, -51.54700538379269403 ) ) ;
#32143=DIRECTION ( 'NONE',  ( 0.000000000000000000, 0.000000000000000000, 1.000000000000000000 ) ) ;
#32206=CARTESIAN_POINT ( 'NONE',  ( -48.47912675150885065, -117.5479369270332057, 15.00000000000000711 ) ) ;
#32218=PLANE ( 'NONE',  #30004 ) ;
#32242=DIRECTION ( 'NONE',  ( -1.000000000000000000, 0.000000000000000000, 0.000000000000000000 ) ) ;
#32535=( LENGTH_UNIT ( ) NAMED_UNIT ( * ) SI_UNIT ( .MILLI., .METRE. ) );
#32694=DIRECTION ( 'NONE',  ( 1.000000000000000000, 0.000000000000000000, -0.000000000000000000 ) ) ;
#32778=EDGE_CURVE ( 'NONE', #15315, #16523, #44923, .T. ) ;
#32808=DIRECTION ( 'NONE',  ( -1.000000000000000000, -0.000000000000000000, -0.000000000000000000 ) ) ;
#32826=DIRECTION ( 'NONE',  ( 1.000000000000000000, 0.000000000000000000, 0.000000000000000000 ) ) ;
#32841=VECTOR ( 'NONE', #32242, 1000.000000000000000 ) ;
#32980=VECTOR ( 'NONE', #43737, 1000.000000000000000 ) ;
#33024=DIRECTION ( 'NONE',  ( 1.000000000000000000, 0.000000000000000000, 0.000000000000000000 ) ) ;
#33045=DIRECTION ( 'NONE',  ( 0.000000000000000000, 0.000000000000000000, 1.000000000000000000 ) ) ;
#33239=ORIENTED_EDGE ( 'NONE', *, *, #27742, .F. ) ;
#33258=EDGE_LOOP ( 'NONE', ( #16267, #43069, #15797, #34714 ) ) ;
#33355=ADVANCED_FACE ( 'NONE', ( #35203 ), #47311, .T. ) ;
#33434=DIRECTION ( 'NONE',  ( -1.000000000000000000, 0.000000000000000000, 0.000000000000000000 ) ) ;
#33436=LINE ( 'NONE', #837, #15260 ) ;
#33525=DIRECTION ( 'NONE',  ( 0.000000000000000000, -1.000000000000000000, 0.000000000000000000 ) ) ;
#33527=ORIENTED_EDGE ( 'NONE', *, *, #41312, .F. ) ;
#33780=FACE_OUTER_BOUND ( 'NONE', #35159, .T. ) ;
#33806=ORIENTED_EDGE ( 'NONE', *, *, #41378, .F. ) ;
#33902=ORIENTED_EDGE ( 'NONE', *, *, #25688, .T. ) ;
#33943=ORIENTED_EDGE ( 'NONE', *, *, #15408, .T. ) ;
#33951=DIRECTION ( 'NONE',  ( -1.000000000000000000, -0.000000000000000000, -0.000000000000000000 ) ) ;
#34026=CYLINDRICAL_SURFACE ( 'NONE', #26213, 4.000000000000003553 ) ;
#34043=DIRECTION ( 'NONE',  ( 0.000000000000000000, -1.346129392433909288E-16, 1.000000000000000000 ) ) ;
#34090=VERTEX_POINT ( 'NONE', #1817 ) ;
#34289=CARTESIAN_POINT ( 'NONE',  ( -160.0000000000000284, -123.5000000000000284, -41.63467731922663972 ) ) ;
#34630=PLANE ( 'NONE',  #2228 ) ;
#34675=ORIENTED_EDGE ( 'NONE', *, *, #35903, .F. ) ;
#34714=ORIENTED_EDGE ( 'NONE', *, *, #45658, .T. ) ;
#34812=FACE_BOUND ( 'NONE', #44129, .T. ) ;
#34884=VECTOR ( 'NONE', #25776, 1000.000000000000000 ) ;
#34984=EDGE_CURVE ( 'NONE', #1807, #50561, #42346, .T. ) ;
#35065=DIRECTION ( 'NONE',  ( 0.000000000000000000, 0.000000000000000000, 1.000000000000000000 ) ) ;
#35122=VECTOR ( 'NONE', #22648, 1000.000000000000000 ) ;
#35159=EDGE_LOOP ( 'NONE', ( #812, #35665, #51696, #17887 ) ) ;
#35203=FACE_OUTER_BOUND ( 'NONE', #44485, .T. ) ;
#35257=ORIENTED_EDGE ( 'NONE', *, *, #44635, .F. ) ;
#35273=EDGE_CURVE ( 'NONE', #15315, #21423, #49670, .T. ) ;
#35310=DIRECTION ( 'NONE',  ( 0.000000000000000000, 0.000000000000000000, 1.000000000000000000 ) ) ;
#35429=SURFACE_SIDE_STYLE ('',( #48047 ) ) ;
#35448=CARTESIAN_POINT ( 'NONE',  ( -160.0000000000000284, -123.5000000000000284, -41.63467731922663972 ) ) ;
#35498=LINE ( 'NONE', #51052, #51659 ) ;
#35525=LINE ( 'NONE', #23710, #27738 ) ;
#35641=CARTESIAN_POINT ( 'NONE',  ( -160.0000000000000284, -123.5000000000000284, 41.63467731922665394 ) ) ;
#35665=ORIENTED_EDGE ( 'NONE', *, *, #7325, .F. ) ;
#35723=DIRECTION ( 'NONE',  ( -0.000000000000000000, -1.000000000000000000, -0.000000000000000000 ) ) ;
#35830=DIRECTION ( 'NONE',  ( -1.000000000000000000, 0.000000000000000000, 0.000000000000000000 ) ) ;
#35903=EDGE_CURVE ( 'NONE', #21423, #40951, #7530, .T. ) ;
#35909=AXIS2_PLACEMENT_3D ( 'NONE', #50925, #39067, #51192 ) ;
#35993=DIRECTION ( 'NONE',  ( -0.000000000000000000, 1.000000000000000000, 0.000000000000000000 ) ) ;
#36165=DIRECTION ( 'NONE',  ( 0.000000000000000000, 0.000000000000000000, 1.000000000000000000 ) ) ;
#36238=DIRECTION ( 'NONE',  ( 0.000000000000000000, 0.8660254037844354880, -0.5000000000000054401 ) ) ;
#36240=LINE ( 'NONE', #24175, #46651 ) ;
#36477=VECTOR ( 'NONE', #33951, 1000.000000000000000 ) ;
#36582=MANIFOLD_SOLID_BREP ( 'Cut-Extrude9', #21210 ) ;
#36677=VECTOR ( 'NONE', #26849, 1000.000000000000227 ) ;
#36759=CARTESIAN_POINT ( 'NONE',  ( -160.0000000000000284, -123.5000000000000284, -37.63467731922663972 ) ) ;
#36793=DIRECTION ( 'NONE',  ( 0.000000000000000000, 0.000000000000000000, -1.000000000000000000 ) ) ;
#36835=VERTEX_POINT ( 'NONE', #13600 ) ;
#36977=VECTOR ( 'NONE', #14550, 1000.000000000000227 ) ;
#37104=LINE ( 'NONE', #17149, #38056 ) ;
#37367=VERTEX_POINT ( 'NONE', #9641 ) ;
#37378=DIRECTION ( 'NONE',  ( 0.000000000000000000, -1.000000000000000000, 0.000000000000000000 ) ) ;
#37606=CARTESIAN_POINT ( 'NONE',  ( -160.0000000000000284, -123.5000000000000284, 41.63467731922665394 ) ) ;
#37797=CARTESIAN_POINT ( 'NONE',  ( -48.47912675150885065, -132.5479369270331915, 6.938893903907228378E-15 ) ) ;
#37823=ORIENTED_EDGE ( 'NONE', *, *, #10451, .F. ) ;
#37876=VECTOR ( 'NONE', #33024, 1000.000000000000000 ) ;
#37956=LINE ( 'NONE', #10106, #7274 ) ;
#37982=VERTEX_POINT ( 'NONE', #21023 ) ;
#38006=VERTEX_POINT ( 'NONE', #1037 ) ;
#38020=ORIENTED_EDGE ( 'NONE', *, *, #31386, .F. ) ;
#38034=CARTESIAN_POINT ( 'NONE',  ( -170.0000000000000284, -113.5000000000000000, 60.00000000000000711 ) ) ;
#38056=VECTOR ( 'NONE', #21079, 1000.000000000000000 ) ;
#38162=DIRECTION ( 'NONE',  ( -1.000000000000000000, 0.000000000000000000, 0.000000000000000000 ) ) ;
#38291=ORIENTED_EDGE ( 'NONE', *, *, #11182, .T. ) ;
#38494=UNCERTAINTY_MEASURE_WITH_UNIT (LENGTH_MEASURE( 1.000000000000000082E-05 ), #51007, 'distance_accuracy_value', 'NONE');
#38579=ORIENTED_EDGE ( 'NONE', *, *, #12967, .T. ) ;
#38678=ORIENTED_EDGE ( 'NONE', *, *, #11182, .F. ) ;
#38697=ORIENTED_EDGE ( 'NONE', *, *, #7675, .T. ) ;
#38758=CARTESIAN_POINT ( 'NONE',  ( -108.4791267515088435, -132.5479369270331915, -186.7953921478704729 ) ) ;
#38768=ORIENTED_EDGE ( 'NONE', *, *, #45193, .T. ) ;
#38791=VECTOR ( 'NONE', #9950, 1000.000000000000000 ) ;
#38897=EDGE_CURVE ( 'NONE', #26043, #18024, #17998, .T. ) ;
#39027=EDGE_LOOP ( 'NONE', ( #41170, #1706, #33527, #7786 ) ) ;
#39067=DIRECTION ( 'NONE',  ( -0.000000000000000000, 1.000000000000000000, 0.000000000000000000 ) ) ;
#39090=DIRECTION ( 'NONE',  ( 0.000000000000000000, 0.000000000000000000, 1.000000000000000000 ) ) ;
#39114=DIRECTION ( 'NONE',  ( 0.000000000000000000, -1.000000000000000000, 0.000000000000000000 ) ) ;
#39466=EDGE_LOOP ( 'NONE', ( #31524, #38579, #39848, #1394 ) ) ;
#39503=CARTESIAN_POINT ( 'NONE',  ( -170.0000000000000284, -113.5000000000000142, 39.99999999999998579 ) ) ;
#39563=CARTESIAN_POINT ( 'NONE',  ( -170.0000000000000284, -173.5000000000000284, -60.00000000000001421 ) ) ;
#39571=ORIENTED_EDGE ( 'NONE', *, *, #48077, .F. ) ;
#39618=VECTOR ( 'NONE', #17672, 1000.000000000000000 ) ;
#39780=VERTEX_POINT ( 'NONE', #17802 ) ;
#39848=ORIENTED_EDGE ( 'NONE', *, *, #46249, .F. ) ;
#39934=EDGE_CURVE ( 'NONE', #31030, #50099, #7009, .T. ) ;
#40019=VERTEX_POINT ( 'NONE', #47989 ) ;
#40061=ADVANCED_FACE ( 'NONE', ( #9599 ), #34026, .F. ) ;
#40067=ORIENTED_EDGE ( 'NONE', *, *, #16347, .T. ) ;
#40171=FACE_OUTER_BOUND ( 'NONE', #39027, .T. ) ;
#40177=MECHANICAL_DESIGN_GEOMETRIC_PRESENTATION_REPRESENTATION('',(#7446),#9970);
#40181=SHAPE_REPRESENTATION ( 'Lockable Linear Guide', ( #31742 ), #8256 ) ;
#40264=EDGE_LOOP ( 'NONE', ( #23149, #38697, #21944, #37823 ) ) ;
#40290=EDGE_CURVE ( 'NONE', #36835, #43044, #44687, .T. ) ;
#40332=LINE ( 'NONE', #20119, #16778 ) ;
#40357=FACE_OUTER_BOUND ( 'NONE', #10356, .T. ) ;
#40361=EDGE_CURVE ( 'NONE', #26611, #5889, #179, .T. ) ;
#40460=VECTOR ( 'NONE', #19104, 1000.000000000000000 ) ;
#40465=ADVANCED_FACE ( 'NONE', ( #27601, #43631, #31020 ), #7629, .F. ) ;
#40532=ORIENTED_EDGE ( 'NONE', *, *, #5334, .F. ) ;
#40951=VERTEX_POINT ( 'NONE', #7689 ) ;
#41032=ADVANCED_FACE ( 'NONE', ( #45272 ), #48938, .T. ) ;
#41141=ORIENTED_EDGE ( 'NONE', *, *, #5081, .F. ) ;
#41170=ORIENTED_EDGE ( 'NONE', *, *, #21374, .T. ) ;
#41180=ORIENTED_EDGE ( 'NONE', *, *, #31408, .T. ) ;
#41197=ORIENTED_EDGE ( 'NONE', *, *, #34984, .T. ) ;
#41261=DIRECTION ( 'NONE',  ( 0.000000000000000000, 1.000000000000000000, 0.000000000000000000 ) ) ;
#41263=LINE ( 'NONE', #5290, #12399 ) ;
#41312=EDGE_CURVE ( 'NONE', #50099, #37367, #2563, .T. ) ;
#41340=DIRECTION ( 'NONE',  ( 0.000000000000000000, 0.000000000000000000, 1.000000000000000000 ) ) ;
#41362=ORIENTED_EDGE ( 'NONE', *, *, #250, .F. ) ;
#41378=EDGE_CURVE ( 'NONE', #26043, #15315, #29896, .T. ) ;
#41381=VERTEX_POINT ( 'NONE', #6250 ) ;
#41397=PLANE ( 'NONE',  #22303 ) ;
#41411=VECTOR ( 'NONE', #18842, 1000.000000000000000 ) ;
#41423=CIRCLE ( 'NONE', #49017, 15.00000000000000000 ) ;
#41553=DIRECTION ( 'NONE',  ( -0.000000000000000000, -0.000000000000000000, 1.000000000000000000 ) ) ;
#41748=VECTOR ( 'NONE', #28278, 1000.000000000000000 ) ;
#41772=CIRCLE ( 'NONE', #45991, 15.00000000000000000 ) ;
#41780=ADVANCED_FACE ( 'NONE', ( #45881 ), #9873, .T. ) ;
#41843=ORIENTED_EDGE ( 'NONE', *, *, #3702, .F. ) ;
#41912=CARTESIAN_POINT ( 'NONE',  ( -170.0000000000000284, -123.5000000000000284, -41.63467731922663972 ) ) ;
#41965=CARTESIAN_POINT ( 'NONE',  ( -160.0000000000000284, -123.5000000000000284, -41.63467731922663972 ) ) ;
#42115=CARTESIAN_POINT ( 'NONE',  ( -170.0000000000000284, -93.50000000000001421, -51.54700538379269403 ) ) ;
#42225=CARTESIAN_POINT ( 'NONE',  ( 60.00000000000001421, -93.50000000000002842, 51.54700538379266561 ) ) ;
#42233=DIRECTION ( 'NONE',  ( -0.000000000000000000, -0.000000000000000000, 1.000000000000000000 ) ) ;
#42346=LINE ( 'NONE', #51283, #35122 ) ;
#42471=AXIS2_PLACEMENT_3D ( 'NONE', #35448, #31510, #11550 ) ;
#42509=VECTOR ( 'NONE', #16693, 1000.000000000000000 ) ;
#42516=DIRECTION ( 'NONE',  ( 0.000000000000000000, 1.000000000000000000, 0.000000000000000000 ) ) ;
#42576=ORIENTED_EDGE ( 'NONE', *, *, #15999, .T. ) ;
#42696=UNCERTAINTY_MEASURE_WITH_UNIT (LENGTH_MEASURE( 1.000000000000000082E-05 ), #32535, 'distance_accuracy_value', 'NONE');
#42751=ADVANCED_FACE ( 'NONE', ( #40357 ), #1479, .T. ) ;
#43044=VERTEX_POINT ( 'NONE', #16154 ) ;
#43069=ORIENTED_EDGE ( 'NONE', *, *, #13139, .F. ) ;
#43230=AXIS2_PLACEMENT_3D ( 'NONE', #20385, #4117, #24335 ) ;
#43239=AXIS2_PLACEMENT_3D ( 'NONE', #3126, #39114, #3379 ) ;
#43401=ORIENTED_EDGE ( 'NONE', *, *, #7675, .F. ) ;
#43619=VERTEX_POINT ( 'NONE', #48933 ) ;
#43631=FACE_BOUND ( 'NONE', #26387, .T. ) ;
#43660=CARTESIAN_POINT ( 'NONE',  ( -170.0000000000000284, -93.50000000000002842, 51.54700538379266561 ) ) ;
#43737=DIRECTION ( 'NONE',  ( 1.000000000000000000, 0.000000000000000000, 0.000000000000000000 ) ) ;
#43775=DIRECTION ( 'NONE',  ( 1.000000000000000000, 0.000000000000000000, 0.000000000000000000 ) ) ;
#43822=EDGE_CURVE ( 'NONE', #45007, #19578, #47061, .T. ) ;
#44129=EDGE_LOOP ( 'NONE', ( #28594, #41180 ) ) ;
#44352=CARTESIAN_POINT ( 'NONE',  ( -170.0000000000000284, -173.5000000000000284, 60.00000000000000000 ) ) ;
#44373=PRODUCT_DEFINITION ( 'UNKNOWN', '', #6621, #29563 ) ;
#44423=CYLINDRICAL_SURFACE ( 'NONE', #2728, 15.00000000000000000 ) ;
#44469=DIRECTION ( 'NONE',  ( 0.000000000000000000, -1.000000000000000000, 0.000000000000000000 ) ) ;
#44485=EDGE_LOOP ( 'NONE', ( #12534, #25833, #13096, #24506 ) ) ;
#44546=CARTESIAN_POINT ( 'NONE',  ( -170.0000000000000284, -113.5000000000000142, 39.99999999999998579 ) ) ;
#44635=EDGE_CURVE ( 'NONE', #15096, #39780, #6884, .T. ) ;
#44687=CIRCLE ( 'NONE', #12783, 4.000000000000003553 ) ;
#44796=APPLICATION_CONTEXT ( 'automotive_design' ) ;
#44834=CARTESIAN_POINT ( 'NONE',  ( -170.0000000000000284, -173.5000000000000284, -60.00000000000001421 ) ) ;
#44853=AXIS2_PLACEMENT_3D ( 'NONE', #13767, #32694, #20887 ) ;
#44884=AXIS2_PLACEMENT_3D ( 'NONE', #7608, #35993, #20214 ) ;
#44923=LINE ( 'NONE', #21009, #22330 ) ;
#45007=VERTEX_POINT ( 'NONE', #49632 ) ;
#45125=CARTESIAN_POINT ( 'NONE',  ( -170.0000000000000284, -113.5000000000000142, -60.00000000000001421 ) ) ;
#45193=EDGE_CURVE ( 'NONE', #37367, #46084, #50161, .T. ) ;
#45249=LINE ( 'NONE', #9235, #34884 ) ;
#45272=FACE_OUTER_BOUND ( 'NONE', #17555, .T. ) ;
#45355=DIRECTION ( 'NONE',  ( -1.000000000000000000, -0.000000000000000000, -0.000000000000000000 ) ) ;
#45413=DIRECTION ( 'NONE',  ( -1.000000000000000000, 0.000000000000000000, 0.000000000000000000 ) ) ;
#45568=CYLINDRICAL_SURFACE ( 'NONE', #443, 4.000000000000003553 ) ;
#45628=CARTESIAN_POINT ( 'NONE',  ( -170.0000000000000284, -93.50000000000001421, -51.54700538379269403 ) ) ;
#45650=EDGE_LOOP ( 'NONE', ( #47096, #90, #2339, #12593 ) ) ;
#45658=EDGE_CURVE ( 'NONE', #24439, #31941, #47427, .T. ) ;
#45687=CARTESIAN_POINT ( 'NONE',  ( -48.47912675150885065, -117.5479369270332057, 6.938893903907228378E-15 ) ) ;
#45812=DIRECTION ( 'NONE',  ( 0.000000000000000000, 0.000000000000000000, 1.000000000000000000 ) ) ;
#45863=CARTESIAN_POINT ( 'NONE',  ( -170.0000000000000284, -93.50000000000002842, 51.54700538379266561 ) ) ;
#45881=FACE_OUTER_BOUND ( 'NONE', #33258, .T. ) ;
#45933=ORIENTED_EDGE ( 'NONE', *, *, #27131, .T. ) ;
#45991=AXIS2_PLACEMENT_3D ( 'NONE', #45687, #5755, #21770 ) ;
#46084=VERTEX_POINT ( 'NONE', #27830 ) ;
#46137=ADVANCED_FACE ( 'NONE', ( #31521 ), #8136, .T. ) ;
#46215=CARTESIAN_POINT ( 'NONE',  ( -108.4791267515088435, -132.5479369270331915, 60.00000000000002132 ) ) ;
#46242=CARTESIAN_POINT ( 'NONE',  ( 60.00000000000001421, -113.5000000000000000, 60.00000000000000711 ) ) ;
#46249=EDGE_CURVE ( 'NONE', #38006, #41381, #41423, .T. ) ;
#46575=PLANE ( 'NONE',  #6492 ) ;
#46598=CIRCLE ( 'NONE', #49930, 4.000000000000003553 ) ;
#46643=DIRECTION ( 'NONE',  ( 1.000000000000000000, 0.000000000000000000, 0.000000000000000000 ) ) ;
#46651=VECTOR ( 'NONE', #35723, 1000.000000000000000 ) ;
#46766=FACE_OUTER_BOUND ( 'NONE', #45650, .T. ) ;
#46973=DIRECTION ( 'NONE',  ( 0.000000000000000000, 6.938893903907222461E-16, 1.000000000000000000 ) ) ;
#47012=LINE ( 'NONE', #6556, #13697 ) ;
#47061=LINE ( 'NONE', #15253, #47929 ) ;
#47066=CARTESIAN_POINT ( 'NONE',  ( -170.0000000000000284, 0.000000000000000000, 0.000000000000000000 ) ) ;
#47096=ORIENTED_EDGE ( 'NONE', *, *, #12967, .F. ) ;
#47174=CARTESIAN_POINT ( 'NONE',  ( -48.47912675150885065, -117.5479369270332057, 15.00000000000000711 ) ) ;
#47203=VECTOR ( 'NONE', #42233, 1000.000000000000000 ) ;
#47273=LINE ( 'NONE', #11244, #31273 ) ;
#47311=PLANE ( 'NONE',  #25714 ) ;
#47384=DIRECTION ( 'NONE',  ( 0.000000000000000000, -1.000000000000000000, 0.000000000000000000 ) ) ;
#47427=LINE ( 'NONE', #31385, #32980 ) ;
#47480=ORIENTED_EDGE ( 'NONE', *, *, #44635, .T. ) ;
#47715=ORIENTED_EDGE ( 'NONE', *, *, #51384, .T. ) ;
#47929=VECTOR ( 'NONE', #31268, 1000.000000000000000 ) ;
#47989=CARTESIAN_POINT ( 'NONE',  ( -160.0000000000000284, -123.5000000000000284, -37.63467731922663972 ) ) ;
#48010=CARTESIAN_POINT ( 'NONE',  ( 60.00000000000001421, -113.5000000000000142, 39.99999999999998579 ) ) ;
#48045=VECTOR ( 'NONE', #19981, 1000.000000000000000 ) ;
#48047=SURFACE_STYLE_FILL_AREA ( #16000 ) ;
#48064=CARTESIAN_POINT ( 'NONE',  ( 11.52087324849114580, -173.5000000000000284, -186.7953921478704729 ) ) ;
#48077=EDGE_CURVE ( 'NONE', #40019, #6739, #21431, .T. ) ;
#48078=( NAMED_UNIT ( * ) PLANE_ANGLE_UNIT ( ) SI_UNIT ( $, .RADIAN. ) );
#48161=DIRECTION ( 'NONE',  ( 0.000000000000000000, -1.346129392433909288E-16, 1.000000000000000000 ) ) ;
#48332=EDGE_CURVE ( 'NONE', #31941, #18024, #45249, .T. ) ;
#48619=EDGE_LOOP ( 'NONE', ( #15870, #3357, #1447, #33806, #29694, #8032, #12079, #19675 ) ) ;
#48674=VERTEX_POINT ( 'NONE', #20209 ) ;
#48689=ADVANCED_FACE ( 'NONE', ( #3149 ), #19429, .F. ) ;
#48815=LINE ( 'NONE', #12539, #32841 ) ;
#48921=ORIENTED_EDGE ( 'NONE', *, *, #5334, .T. ) ;
#48933=CARTESIAN_POINT ( 'NONE',  ( -108.4791267515088435, -132.5479369270331915, -60.00000000000002842 ) ) ;
#48938=PLANE ( 'NONE',  #28791 ) ;
#49017=AXIS2_PLACEMENT_3D ( 'NONE', #37797, #17839, #9692 ) ;
#49177=DIRECTION ( 'NONE',  ( -1.000000000000000000, 0.000000000000000000, 0.000000000000000000 ) ) ;
#49219=ADVANCED_FACE ( 'NONE', ( #1925 ), #45568, .F. ) ;
#49236=AXIS2_PLACEMENT_3D ( 'NONE', #38758, #26157, #13831 ) ;
#49288=ORIENTED_EDGE ( 'NONE', *, *, #10451, .T. ) ;
#49345=ORIENTED_EDGE ( 'NONE', *, *, #51024, .T. ) ;
#49378=ORIENTED_EDGE ( 'NONE', *, *, #31386, .T. ) ;
#49551=DIRECTION ( 'NONE',  ( 1.000000000000000000, 0.000000000000000000, 0.000000000000000000 ) ) ;
#49632=CARTESIAN_POINT ( 'NONE',  ( 60.00000000000001421, -113.5000000000000142, -60.00000000000001421 ) ) ;
#49637=CARTESIAN_POINT ( 'NONE',  ( -108.4791267515088435, -173.5000000000000284, -186.7953921478704729 ) ) ;
#49670=LINE ( 'NONE', #21030, #12503 ) ;
#49719=AXIS2_PLACEMENT_3D ( 'NONE', #336, #4042, #32143 ) ;
#49745=ORIENTED_EDGE ( 'NONE', *, *, #38897, .F. ) ;
#49800=ORIENTED_EDGE ( 'NONE', *, *, #7091, .F. ) ;
#49816=EDGE_CURVE ( 'NONE', #46084, #16523, #36240, .T. ) ;
#49900=DIRECTION ( 'NONE',  ( 0.000000000000000000, -1.156482317317871232E-16, 1.000000000000000000 ) ) ;
#49930=AXIS2_PLACEMENT_3D ( 'NONE', #41912, #35830, #35310 ) ;
#50099=VERTEX_POINT ( 'NONE', #10203 ) ;
#50114=ADVANCED_FACE ( 'NONE', ( #50944 ), #34630, .T. ) ;
#50161=LINE ( 'NONE', #46215, #38791 ) ;
#50296=ORIENTED_EDGE ( 'NONE', *, *, #48332, .T. ) ;
#50408=ORIENTED_EDGE ( 'NONE', *, *, #45193, .F. ) ;
#50466=ADVANCED_FACE ( 'NONE', ( #34812, #9894 ), #25914, .F. ) ;
#50551=LINE ( 'NONE', #6666, #36977 ) ;
#50561=VERTEX_POINT ( 'NONE', #1993 ) ;
#50801=PRODUCT_DEFINITION_SHAPE ( 'NONE', 'NONE',  #44373 ) ;
#50803=CARTESIAN_POINT ( 'NONE',  ( 60.00000000000001421, -113.5000000000000000, -40.00000000000001421 ) ) ;
#50925=CARTESIAN_POINT ( 'NONE',  ( -48.47912675150885065, -117.5479369270332057, 6.938893903907228378E-15 ) ) ;
#50944=FACE_OUTER_BOUND ( 'NONE', #22565, .T. ) ;
#51007=( LENGTH_UNIT ( ) NAMED_UNIT ( * ) SI_UNIT ( .MILLI., .METRE. ) );
#51024=EDGE_CURVE ( 'NONE', #21423, #51701, #12368, .T. ) ;
#51052=CARTESIAN_POINT ( 'NONE',  ( -170.0000000000000284, -113.5000000000000142, -60.00000000000001421 ) ) ;
#51192=DIRECTION ( 'NONE',  ( 0.000000000000000000, -0.000000000000000000, 1.000000000000000000 ) ) ;
#51283=CARTESIAN_POINT ( 'NONE',  ( 60.00000000000001421, -173.5000000000000284, 60.00000000000000000 ) ) ;
#51384=EDGE_CURVE ( 'NONE', #48674, #21917, #1976, .T. ) ;
#51406=AXIS2_PLACEMENT_3D ( 'NONE', #5939, #21953, #26403 ) ;
#51518=ORIENTED_EDGE ( 'NONE', *, *, #40361, .F. ) ;
#51659=VECTOR ( 'NONE', #19472, 1000.000000000000000 ) ;
#51696=ORIENTED_EDGE ( 'NONE', *, *, #7670, .T. ) ;
#51701=VERTEX_POINT ( 'NONE', #4565 ) ;
#51717=CIRCLE ( 'NONE', #3040, 4.000000000000003553 ) ;
#51743=( NAMED_UNIT ( * ) SI_UNIT ( $, .STERADIAN. ) SOLID_ANGLE_UNIT ( ) );
#51851=DIRECTION ( 'NONE',  ( 0.000000000000000000, 6.938893903907229364E-16, 1.000000000000000000 ) ) ;
#51990=VECTOR ( 'NONE', #43775, 1000.000000000000000 ) ;
#52015=ORIENTED_EDGE ( 'NONE', *, *, #16405, .T. ) ;
ENDSEC;
END-ISO-10303-21;
